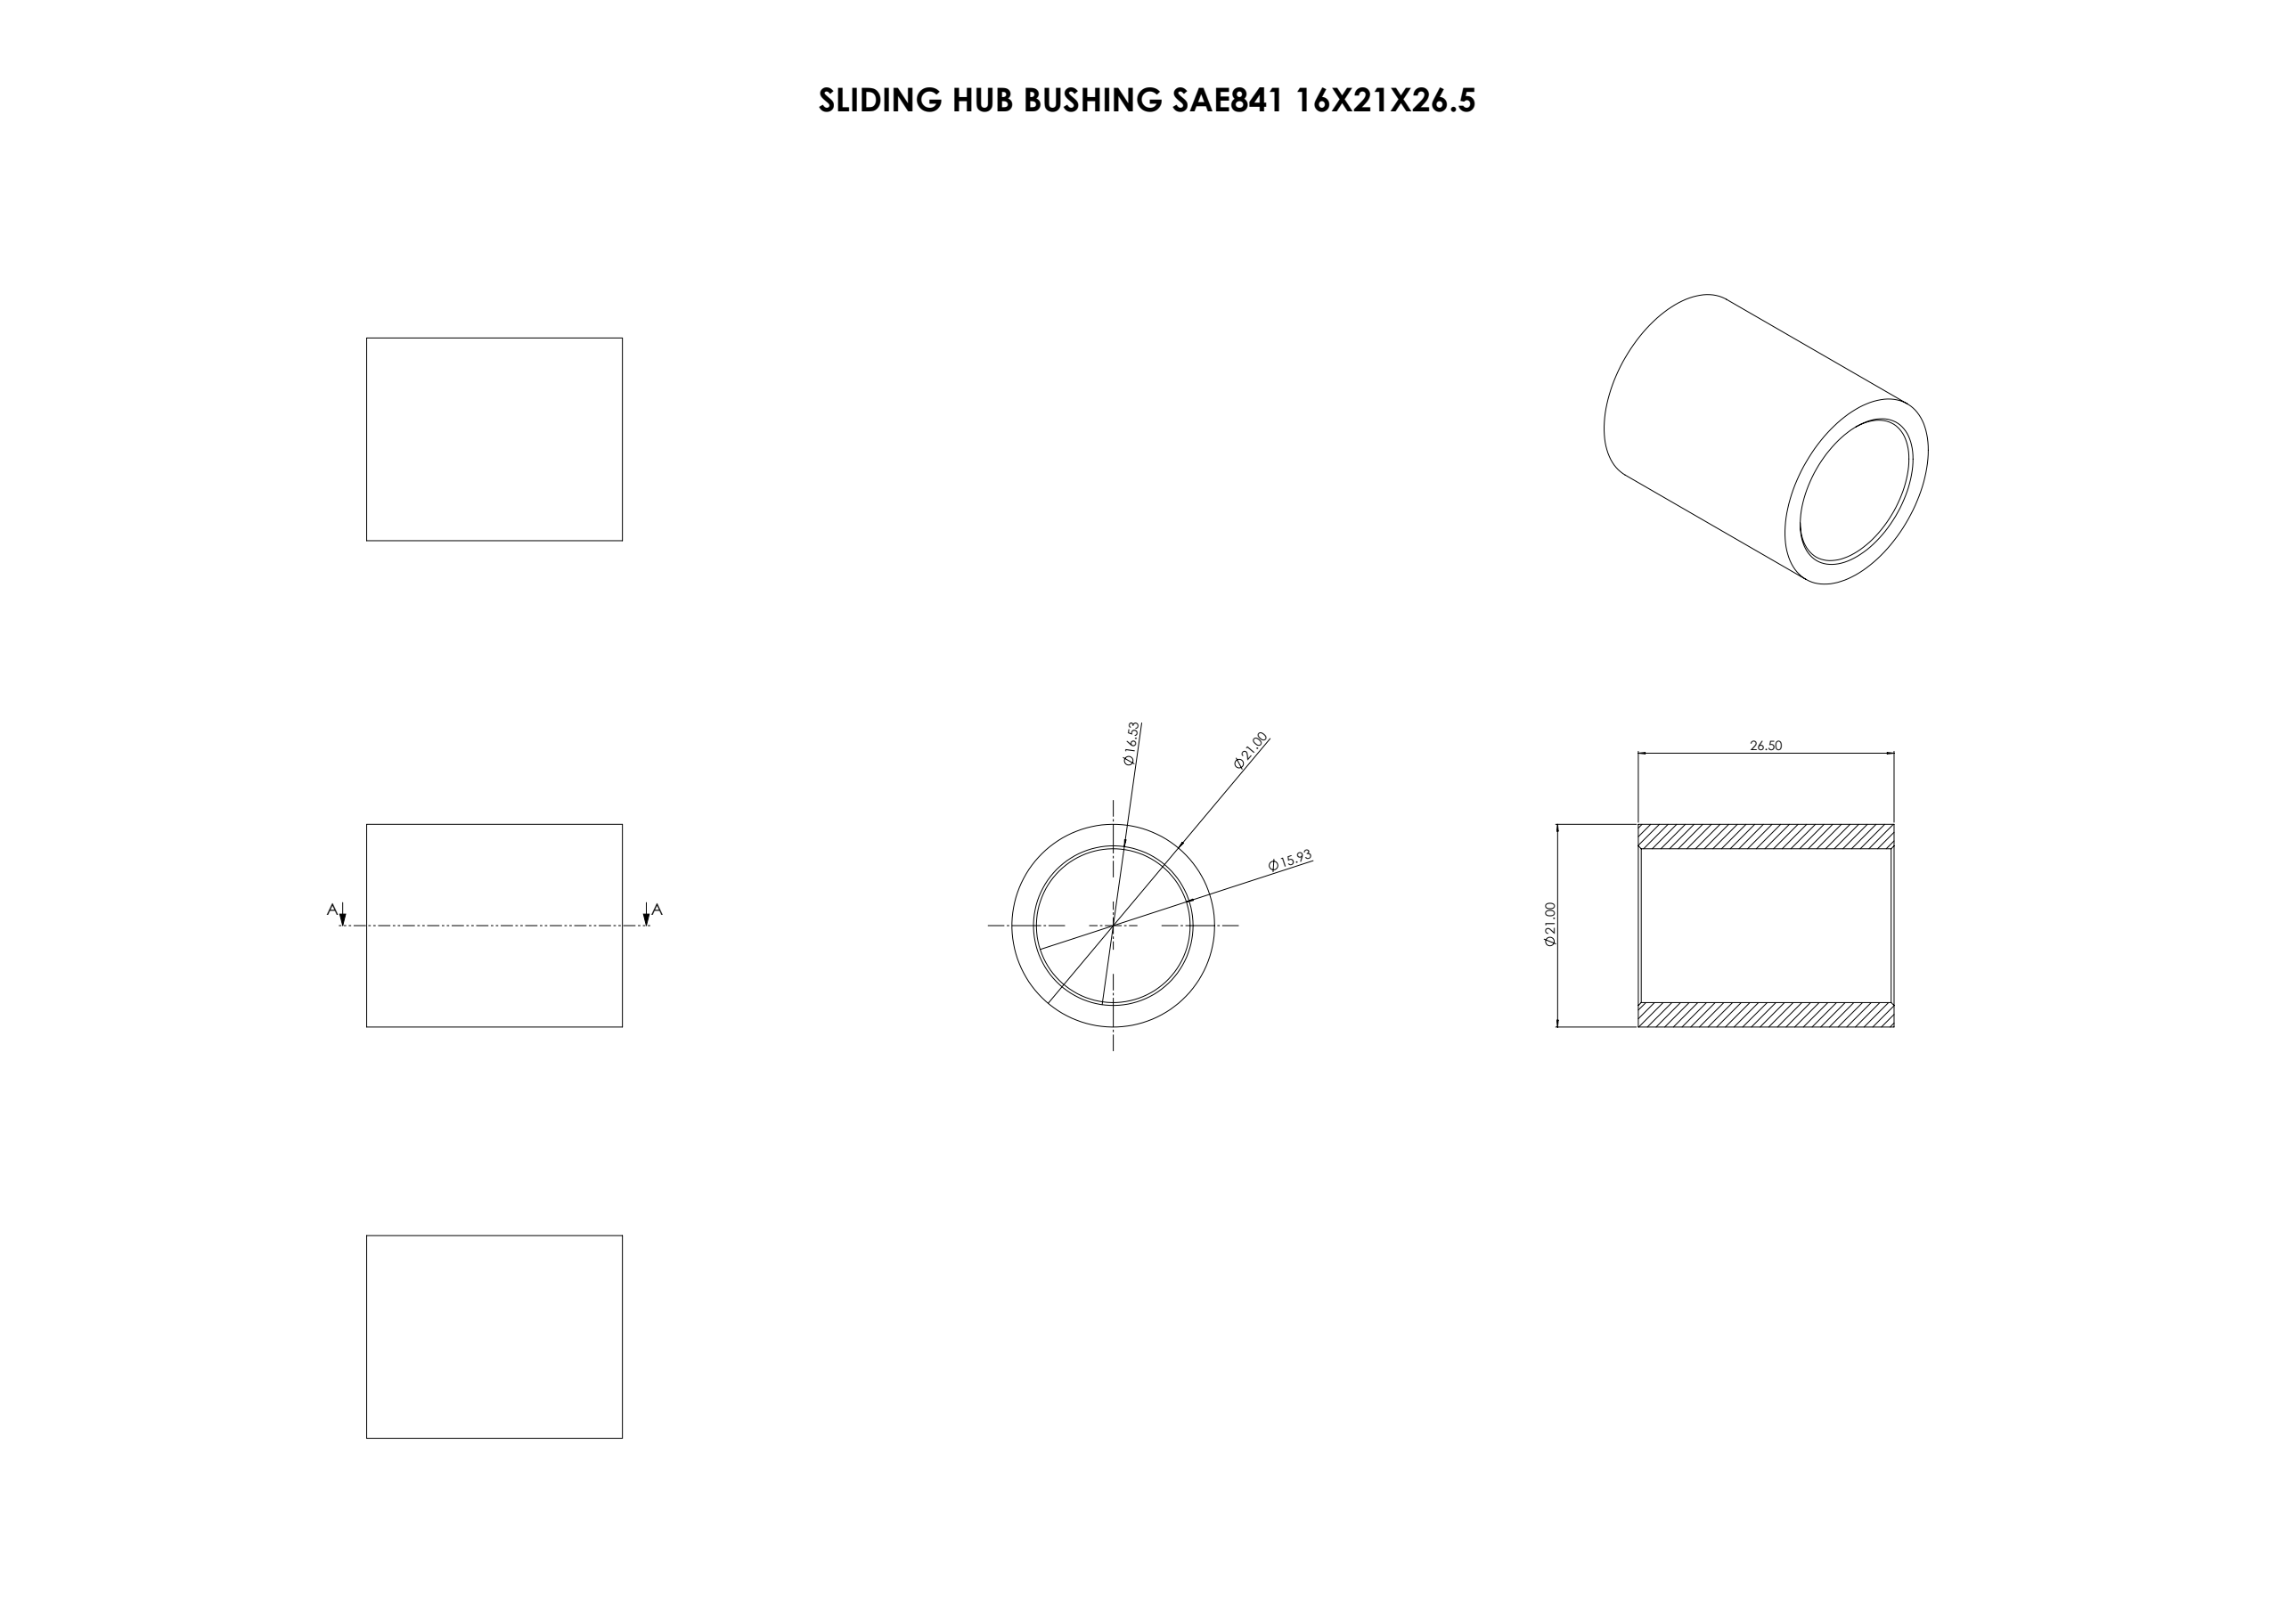
ISO-10303-21;
HEADER;
/* Generated by software containing ST-Developer
 * from STEP Tools, Inc. (www.steptools.com) 
 */

FILE_DESCRIPTION(
/* description */ (''),
/* implementation_level */ '2;1');

FILE_NAME(
/* name */ '07_Sliding_Hub_Bushing_SAE841_16x21x26.5.step',
/* time_stamp */ '2026-10-24T13:41:11-07:00',
/* author */ (''),
/* organization */ (''),
/* preprocessor_version */ 'ST-DEVELOPER v20.2',
/* originating_system */ 'Autodesk Translation Framework v15.15.0.0',
/* authorisation */ '');

FILE_SCHEMA (('AUTOMOTIVE_DESIGN { 1 0 10303 214 3 1 1 }'));
ENDSEC;

DATA;
#10=MECHANICAL_DESIGN_GEOMETRIC_PRESENTATION_REPRESENTATION('',(#127),#12813);
#97=CONICAL_SURFACE('',#4923,8.115,0.785398163397445);
#98=CONICAL_SURFACE('',#4927,8.115,0.785398163397448);
#107=SHAPE_REPRESENTATION_RELATIONSHIP('SRR','None',#12860,#117);
#117=ADVANCED_BREP_SHAPE_REPRESENTATION('',(#137),#12809);
#127=STYLED_ITEM('',(#12967),#137);
#137=MANIFOLD_SOLID_BREP('Body1',#4390);
#161=FACE_BOUND('',#836,.T.);
#162=FACE_BOUND('',#841,.T.);
#220=PLANE('',#4921);
#221=PLANE('',#4929);
#544=FACE_OUTER_BOUND('',#834,.T.);
#545=FACE_OUTER_BOUND('',#835,.T.);
#546=FACE_OUTER_BOUND('',#837,.T.);
#547=FACE_OUTER_BOUND('',#838,.T.);
#548=FACE_OUTER_BOUND('',#839,.T.);
#549=FACE_OUTER_BOUND('',#840,.T.);
#834=EDGE_LOOP('',(#3833,#3834,#3835,#3836));
#835=EDGE_LOOP('',(#3837));
#836=EDGE_LOOP('',(#3838));
#837=EDGE_LOOP('',(#3839,#3840,#3841,#3842));
#838=EDGE_LOOP('',(#3843,#3844,#3845,#3846));
#839=EDGE_LOOP('',(#3847,#3848,#3849,#3850));
#840=EDGE_LOOP('',(#3851));
#841=EDGE_LOOP('',(#3852));
#1103=CIRCLE('',#4919,10.5);
#1104=CIRCLE('',#4920,10.5);
#1105=CIRCLE('',#4922,8.265);
#1106=CIRCLE('',#4924,7.965);
#1107=CIRCLE('',#4926,7.965);
#1108=CIRCLE('',#4928,8.265);
#1275=LINE('',#12574,#1505);
#1276=LINE('',#12581,#1506);
#1277=LINE('',#12585,#1507);
#1278=LINE('',#12589,#1508);
#1505=VECTOR('',#5986,10.5);
#1506=VECTOR('',#5995,8.115);
#1507=VECTOR('',#6000,7.965);
#1508=VECTOR('',#6005,8.115);
#2080=VERTEX_POINT('',#12571);
#2081=VERTEX_POINT('',#12573);
#2082=VERTEX_POINT('',#12577);
#2083=VERTEX_POINT('',#12580);
#2084=VERTEX_POINT('',#12584);
#2085=VERTEX_POINT('',#12588);
#2669=EDGE_CURVE('',#2080,#2080,#1103,.T.);
#2670=EDGE_CURVE('',#2080,#2081,#1275,.T.);
#2671=EDGE_CURVE('',#2081,#2081,#1104,.T.);
#2672=EDGE_CURVE('',#2082,#2082,#1105,.T.);
#2673=EDGE_CURVE('',#2082,#2083,#1276,.T.);
#2674=EDGE_CURVE('',#2083,#2083,#1106,.T.);
#2675=EDGE_CURVE('',#2083,#2084,#1277,.T.);
#2676=EDGE_CURVE('',#2084,#2084,#1107,.T.);
#2677=EDGE_CURVE('',#2084,#2085,#1278,.T.);
#2678=EDGE_CURVE('',#2085,#2085,#1108,.T.);
#3833=ORIENTED_EDGE('',*,*,#2669,.F.);
#3834=ORIENTED_EDGE('',*,*,#2670,.T.);
#3835=ORIENTED_EDGE('',*,*,#2671,.T.);
#3836=ORIENTED_EDGE('',*,*,#2670,.F.);
#3837=ORIENTED_EDGE('',*,*,#2669,.T.);
#3838=ORIENTED_EDGE('',*,*,#2672,.F.);
#3839=ORIENTED_EDGE('',*,*,#2672,.T.);
#3840=ORIENTED_EDGE('',*,*,#2673,.T.);
#3841=ORIENTED_EDGE('',*,*,#2674,.F.);
#3842=ORIENTED_EDGE('',*,*,#2673,.F.);
#3843=ORIENTED_EDGE('',*,*,#2674,.T.);
#3844=ORIENTED_EDGE('',*,*,#2675,.T.);
#3845=ORIENTED_EDGE('',*,*,#2676,.F.);
#3846=ORIENTED_EDGE('',*,*,#2675,.F.);
#3847=ORIENTED_EDGE('',*,*,#2676,.T.);
#3848=ORIENTED_EDGE('',*,*,#2677,.T.);
#3849=ORIENTED_EDGE('',*,*,#2678,.F.);
#3850=ORIENTED_EDGE('',*,*,#2677,.F.);
#3851=ORIENTED_EDGE('',*,*,#2671,.F.);
#3852=ORIENTED_EDGE('',*,*,#2678,.T.);
#4106=CYLINDRICAL_SURFACE('',#4918,10.5);
#4107=CYLINDRICAL_SURFACE('',#4925,7.965);
#4334=ADVANCED_FACE('',(#544),#4106,.T.);
#4335=ADVANCED_FACE('',(#545,#161),#220,.T.);
#4336=ADVANCED_FACE('',(#546),#97,.F.);
#4337=ADVANCED_FACE('',(#547),#4107,.F.);
#4338=ADVANCED_FACE('',(#548),#98,.F.);
#4339=ADVANCED_FACE('',(#549,#162),#221,.T.);
#4390=CLOSED_SHELL('',(#4334,#4335,#4336,#4337,#4338,#4339));
#4917=AXIS2_PLACEMENT_3D('',#12569,#5980,#5981);
#4918=AXIS2_PLACEMENT_3D('',#12570,#5982,#5983);
#4919=AXIS2_PLACEMENT_3D('',#12572,#5984,#5985);
#4920=AXIS2_PLACEMENT_3D('',#12575,#5987,#5988);
#4921=AXIS2_PLACEMENT_3D('',#12576,#5989,#5990);
#4922=AXIS2_PLACEMENT_3D('',#12578,#5991,#5992);
#4923=AXIS2_PLACEMENT_3D('',#12579,#5993,#5994);
#4924=AXIS2_PLACEMENT_3D('',#12582,#5996,#5997);
#4925=AXIS2_PLACEMENT_3D('',#12583,#5998,#5999);
#4926=AXIS2_PLACEMENT_3D('',#12586,#6001,#6002);
#4927=AXIS2_PLACEMENT_3D('',#12587,#6003,#6004);
#4928=AXIS2_PLACEMENT_3D('',#12590,#6006,#6007);
#4929=AXIS2_PLACEMENT_3D('',#12591,#6008,#6009);
#5980=DIRECTION('axis',(0.,0.,1.));
#5981=DIRECTION('refdir',(1.,0.,0.));
#5982=DIRECTION('center_axis',(1.,0.,0.));
#5983=DIRECTION('ref_axis',(0.,1.,0.));
#5984=DIRECTION('center_axis',(1.,0.,0.));
#5985=DIRECTION('ref_axis',(0.,0.,-1.));
#5986=DIRECTION('',(-1.,0.,0.));
#5987=DIRECTION('center_axis',(1.,0.,0.));
#5988=DIRECTION('ref_axis',(0.,0.,-1.));
#5989=DIRECTION('center_axis',(1.,0.,0.));
#5990=DIRECTION('ref_axis',(0.,0.,-1.));
#5991=DIRECTION('center_axis',(1.,0.,0.));
#5992=DIRECTION('ref_axis',(0.,0.,-1.));
#5993=DIRECTION('center_axis',(1.,0.,0.));
#5994=DIRECTION('ref_axis',(0.,1.,0.));
#5995=DIRECTION('',(-0.70710678118655,0.707106781186545,8.6595605623549E-17));
#5996=DIRECTION('center_axis',(1.,0.,0.));
#5997=DIRECTION('ref_axis',(0.,0.,-1.));
#5998=DIRECTION('center_axis',(1.,0.,0.));
#5999=DIRECTION('ref_axis',(0.,1.,0.));
#6000=DIRECTION('',(-1.,0.,0.));
#6001=DIRECTION('center_axis',(1.,0.,0.));
#6002=DIRECTION('ref_axis',(0.,0.,-1.));
#6003=DIRECTION('center_axis',(-1.,0.,0.));
#6004=DIRECTION('ref_axis',(0.,1.,0.));
#6005=DIRECTION('',(-0.707106781186548,-0.707106781186548,-8.65956056235493E-17));
#6006=DIRECTION('center_axis',(1.,0.,0.));
#6007=DIRECTION('ref_axis',(0.,0.,-1.));
#6008=DIRECTION('center_axis',(-1.,0.,0.));
#6009=DIRECTION('ref_axis',(0.,0.,1.));
#12569=CARTESIAN_POINT('',(0.,0.,0.));
#12570=CARTESIAN_POINT('Origin',(28.75,0.,0.));
#12571=CARTESIAN_POINT('',(42.,-10.5,-1.28587913910472E-15));
#12572=CARTESIAN_POINT('Origin',(42.,0.,0.));
#12573=CARTESIAN_POINT('',(15.5,-10.5,-1.28587913910472E-15));
#12574=CARTESIAN_POINT('',(28.75,-10.5,-1.28587913910472E-15));
#12575=CARTESIAN_POINT('Origin',(15.5,0.,0.));
#12576=CARTESIAN_POINT('Origin',(42.,8.265,0.));
#12577=CARTESIAN_POINT('',(42.,-8.265,-1.01217057949529E-15));
#12578=CARTESIAN_POINT('Origin',(42.,0.,0.));
#12579=CARTESIAN_POINT('Origin',(41.85,0.,0.));
#12580=CARTESIAN_POINT('',(41.7,-7.965,-9.75431175520866E-16));
#12581=CARTESIAN_POINT('',(41.85,-8.115,-9.93800877508077E-16));
#12582=CARTESIAN_POINT('Origin',(41.7,0.,0.));
#12583=CARTESIAN_POINT('Origin',(28.75,0.,0.));
#12584=CARTESIAN_POINT('',(15.8,-7.965,-9.75431175520867E-16));
#12585=CARTESIAN_POINT('',(28.75,-7.965,-9.75431175520867E-16));
#12586=CARTESIAN_POINT('Origin',(15.8,0.,0.));
#12587=CARTESIAN_POINT('Origin',(15.65,0.,0.));
#12588=CARTESIAN_POINT('',(15.5,-8.265,-1.01217057949529E-15));
#12589=CARTESIAN_POINT('',(15.65,-8.115,-9.93800877508077E-16));
#12590=CARTESIAN_POINT('Origin',(15.5,0.,0.));
#12591=CARTESIAN_POINT('Origin',(15.5,10.5,0.));
#12797=UNCERTAINTY_MEASURE_WITH_UNIT(LENGTH_MEASURE(0.01),#12814,
'DISTANCE_ACCURACY_VALUE',
'Maximum model space distance between geometric entities at asserted c
onnectivities');
#12801=UNCERTAINTY_MEASURE_WITH_UNIT(LENGTH_MEASURE(0.01),#12814,
'DISTANCE_ACCURACY_VALUE',
'Maximum model space distance between geometric entities at asserted c
onnectivities');
#12809=(
GEOMETRIC_REPRESENTATION_CONTEXT(3)
GLOBAL_UNCERTAINTY_ASSIGNED_CONTEXT((#12797))
GLOBAL_UNIT_ASSIGNED_CONTEXT((#12814,#12816,#12817))
REPRESENTATION_CONTEXT('','3D')
);
#12813=(
GEOMETRIC_REPRESENTATION_CONTEXT(3)
GLOBAL_UNCERTAINTY_ASSIGNED_CONTEXT((#12801))
GLOBAL_UNIT_ASSIGNED_CONTEXT((#12814,#12816,#12817))
REPRESENTATION_CONTEXT('','3D')
);
#12814=(
LENGTH_UNIT()
NAMED_UNIT(*)
SI_UNIT(.MILLI.,.METRE.)
);
#12816=(
NAMED_UNIT(*)
PLANE_ANGLE_UNIT()
SI_UNIT($,.RADIAN.)
);
#12817=(
NAMED_UNIT(*)
SI_UNIT($,.STERADIAN.)
SOLID_ANGLE_UNIT()
);
#12825=SHAPE_DEFINITION_REPRESENTATION(#12836,#12860);
#12836=PRODUCT_DEFINITION_SHAPE('',$,#12872);
#12860=SHAPE_REPRESENTATION('',(#4917),#12809);
#12864=PRODUCT_DEFINITION_CONTEXT('part definition',#12899,'design');
#12872=PRODUCT_DEFINITION('2026-10-11-12-17-36-203',
'07_Sliding_Hub_Bushing_SAE841_16x21x26.5',#12883,#12864);
#12883=PRODUCT_DEFINITION_FORMATION('',$,#12908);
#12899=APPLICATION_CONTEXT(
'Core Data for Automotive Mechanical Design Process');
#12900=PRODUCT_CONTEXT('part definition',#12899,'mechanical');
#12908=PRODUCT('2026-10-11-12-17-36-203',
'07_Sliding_Hub_Bushing_SAE841_16x21x26.5',$,(#12900));
#12961=COLOUR_RGB('Sky Blue',0.24,0.69,0.87);
#12962=FILL_AREA_STYLE_COLOUR('',#12961);
#12963=FILL_AREA_STYLE('',(#12962));
#12964=SURFACE_STYLE_FILL_AREA(#12963);
#12965=SURFACE_SIDE_STYLE('',(#12964));
#12966=SURFACE_STYLE_USAGE(.BOTH.,#12965);
#12967=PRESENTATION_STYLE_ASSIGNMENT((#12966));
ENDSEC;
END-ISO-10303-21;
